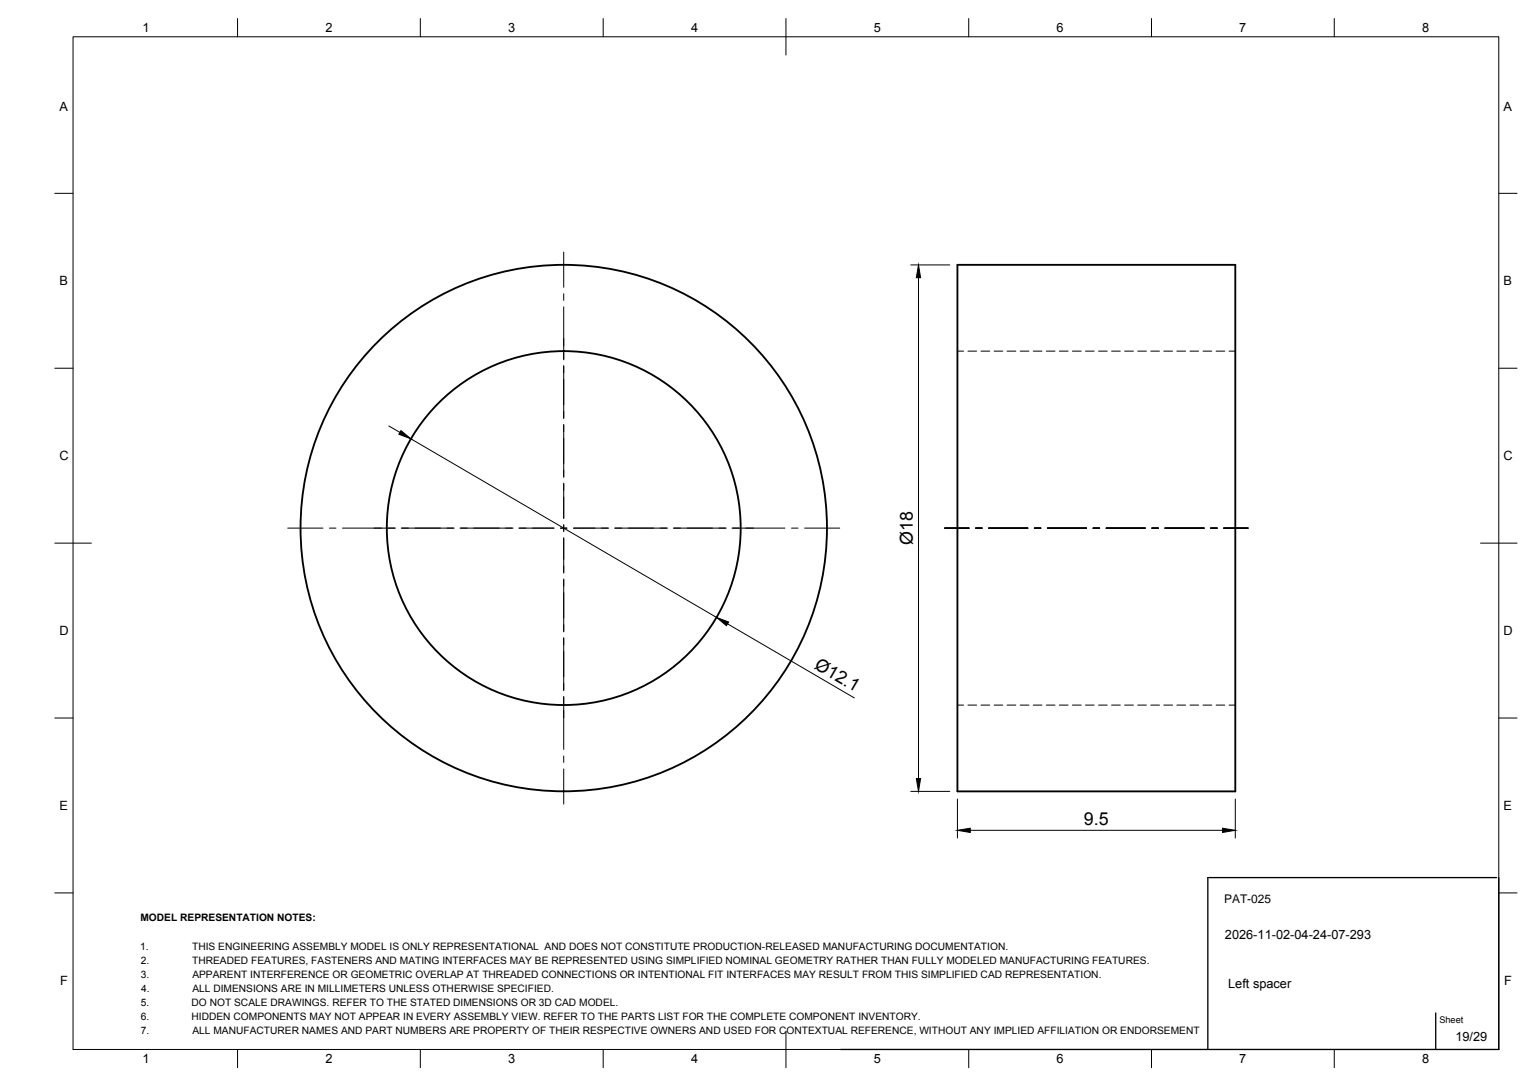
ISO-10303-21;
HEADER;
/* Generated by software containing ST-Developer
 * from STEP Tools, Inc. (www.steptools.com) 
 */

FILE_DESCRIPTION(
/* description */ ('Counter shaft with two pulleys and keyed hub'),
/* implementation_level */ '2;1');

FILE_NAME(
/* name */ 'Left spacer.step',
/* time_stamp */ '2026-10-27T10:46:10-07:00',
/* author */ (''),
/* organization */ (''),
/* preprocessor_version */ 'ST-DEVELOPER v20.2',
/* originating_system */ 'Autodesk Translation Framework v15.17.0.0',
/* authorisation */ '');

FILE_SCHEMA (('AUTOMOTIVE_DESIGN { 1 0 10303 214 3 1 1 }'));
ENDSEC;

DATA;
#10=MECHANICAL_DESIGN_GEOMETRIC_PRESENTATION_REPRESENTATION('',(#303),#10821);
#252=SHAPE_REPRESENTATION_RELATIONSHIP('SRR','None',#10940,#277);
#277=ADVANCED_BREP_SHAPE_REPRESENTATION('',(#328),#10808);
#303=STYLED_ITEM('',(#11149),#328);
#328=MANIFOLD_SOLID_BREP('Body1',#5587);
#395=FACE_BOUND('',#1085,.T.);
#396=FACE_BOUND('',#1087,.T.);
#515=PLANE('',#6121);
#516=PLANE('',#6122);
#713=FACE_OUTER_BOUND('',#1082,.T.);
#714=FACE_OUTER_BOUND('',#1083,.T.);
#715=FACE_OUTER_BOUND('',#1084,.T.);
#716=FACE_OUTER_BOUND('',#1086,.T.);
#1082=EDGE_LOOP('',(#4159,#4160,#4161,#4162));
#1083=EDGE_LOOP('',(#4163,#4164,#4165,#4166));
#1084=EDGE_LOOP('',(#4167));
#1085=EDGE_LOOP('',(#4168));
#1086=EDGE_LOOP('',(#4169));
#1087=EDGE_LOOP('',(#4170));
#1471=LINE('',#9333,#1860);
#1472=LINE('',#9339,#1861);
#1860=VECTOR('',#7203,0.605);
#1861=VECTOR('',#7210,0.9);
#2162=CIRCLE('',#6116,0.605);
#2163=CIRCLE('',#6117,0.605);
#2164=CIRCLE('',#6119,0.9);
#2165=CIRCLE('',#6120,0.9);
#2567=VERTEX_POINT('',#9330);
#2568=VERTEX_POINT('',#9332);
#2569=VERTEX_POINT('',#9336);
#2570=VERTEX_POINT('',#9338);
#3152=EDGE_CURVE('',#2567,#2567,#2162,.T.);
#3153=EDGE_CURVE('',#2567,#2568,#1471,.T.);
#3154=EDGE_CURVE('',#2568,#2568,#2163,.T.);
#3155=EDGE_CURVE('',#2569,#2569,#2164,.T.);
#3156=EDGE_CURVE('',#2569,#2570,#1472,.T.);
#3157=EDGE_CURVE('',#2570,#2570,#2165,.T.);
#4159=ORIENTED_EDGE('',*,*,#3152,.F.);
#4160=ORIENTED_EDGE('',*,*,#3153,.T.);
#4161=ORIENTED_EDGE('',*,*,#3154,.T.);
#4162=ORIENTED_EDGE('',*,*,#3153,.F.);
#4163=ORIENTED_EDGE('',*,*,#3155,.F.);
#4164=ORIENTED_EDGE('',*,*,#3156,.T.);
#4165=ORIENTED_EDGE('',*,*,#3157,.T.);
#4166=ORIENTED_EDGE('',*,*,#3156,.F.);
#4167=ORIENTED_EDGE('',*,*,#3155,.T.);
#4168=ORIENTED_EDGE('',*,*,#3152,.T.);
#4169=ORIENTED_EDGE('',*,*,#3157,.F.);
#4170=ORIENTED_EDGE('',*,*,#3154,.F.);
#5149=CYLINDRICAL_SURFACE('',#6115,0.605);
#5150=CYLINDRICAL_SURFACE('',#6118,0.9);
#5384=ADVANCED_FACE('',(#713),#5149,.F.);
#5385=ADVANCED_FACE('',(#714),#5150,.T.);
#5386=ADVANCED_FACE('',(#715,#395),#515,.T.);
#5387=ADVANCED_FACE('',(#716,#396),#516,.F.);
#5587=CLOSED_SHELL('',(#5384,#5385,#5386,#5387));
#6114=AXIS2_PLACEMENT_3D('',#9328,#7197,#7198);
#6115=AXIS2_PLACEMENT_3D('',#9329,#7199,#7200);
#6116=AXIS2_PLACEMENT_3D('',#9331,#7201,#7202);
#6117=AXIS2_PLACEMENT_3D('',#9334,#7204,#7205);
#6118=AXIS2_PLACEMENT_3D('',#9335,#7206,#7207);
#6119=AXIS2_PLACEMENT_3D('',#9337,#7208,#7209);
#6120=AXIS2_PLACEMENT_3D('',#9340,#7211,#7212);
#6121=AXIS2_PLACEMENT_3D('',#9341,#7213,#7214);
#6122=AXIS2_PLACEMENT_3D('',#9342,#7215,#7216);
#7197=DIRECTION('axis',(0.,0.,1.));
#7198=DIRECTION('refdir',(1.,0.,0.));
#7199=DIRECTION('center_axis',(0.,1.,0.));
#7200=DIRECTION('ref_axis',(1.,0.,0.));
#7201=DIRECTION('center_axis',(0.,-1.,0.));
#7202=DIRECTION('ref_axis',(1.,0.,0.));
#7203=DIRECTION('',(0.,-1.,0.));
#7204=DIRECTION('center_axis',(0.,-1.,0.));
#7205=DIRECTION('ref_axis',(1.,0.,0.));
#7206=DIRECTION('center_axis',(0.,1.,0.));
#7207=DIRECTION('ref_axis',(1.,0.,0.));
#7208=DIRECTION('center_axis',(0.,1.,0.));
#7209=DIRECTION('ref_axis',(1.,0.,0.));
#7210=DIRECTION('',(0.,-1.,0.));
#7211=DIRECTION('center_axis',(0.,1.,0.));
#7212=DIRECTION('ref_axis',(1.,0.,0.));
#7213=DIRECTION('center_axis',(0.,1.,0.));
#7214=DIRECTION('ref_axis',(1.,0.,0.));
#7215=DIRECTION('center_axis',(0.,1.,0.));
#7216=DIRECTION('ref_axis',(1.,0.,0.));
#9328=CARTESIAN_POINT('',(0.,0.,0.));
#9329=CARTESIAN_POINT('Origin',(0.,-3.45,4.53));
#9330=CARTESIAN_POINT('',(-0.605,-2.5,4.53));
#9331=CARTESIAN_POINT('Origin',(0.,-2.5,4.53));
#9332=CARTESIAN_POINT('',(-0.605,-3.45,4.53));
#9333=CARTESIAN_POINT('',(-0.605,-3.45,4.53));
#9334=CARTESIAN_POINT('Origin',(0.,-3.45,4.53));
#9335=CARTESIAN_POINT('Origin',(0.,-3.45,4.53));
#9336=CARTESIAN_POINT('',(-0.9,-2.5,4.53));
#9337=CARTESIAN_POINT('Origin',(0.,-2.5,4.53));
#9338=CARTESIAN_POINT('',(-0.9,-3.45,4.53));
#9339=CARTESIAN_POINT('',(-0.9,-3.45,4.53));
#9340=CARTESIAN_POINT('Origin',(0.,-3.45,4.53));
#9341=CARTESIAN_POINT('Origin',(0.,-2.5,4.53));
#9342=CARTESIAN_POINT('Origin',(0.,-3.45,4.53));
#10778=UNCERTAINTY_MEASURE_WITH_UNIT(LENGTH_MEASURE(0.001),#10822,
'DISTANCE_ACCURACY_VALUE',
'Maximum model space distance between geometric entities at asserted c
onnectivities');
#10791=UNCERTAINTY_MEASURE_WITH_UNIT(LENGTH_MEASURE(0.001),#10822,
'DISTANCE_ACCURACY_VALUE',
'Maximum model space distance between geometric entities at asserted c
onnectivities');
#10808=(
GEOMETRIC_REPRESENTATION_CONTEXT(3)
GLOBAL_UNCERTAINTY_ASSIGNED_CONTEXT((#10778))
GLOBAL_UNIT_ASSIGNED_CONTEXT((#10822,#10824,#10825))
REPRESENTATION_CONTEXT('','3D')
);
#10821=(
GEOMETRIC_REPRESENTATION_CONTEXT(3)
GLOBAL_UNCERTAINTY_ASSIGNED_CONTEXT((#10791))
GLOBAL_UNIT_ASSIGNED_CONTEXT((#10822,#10824,#10825))
REPRESENTATION_CONTEXT('','3D')
);
#10822=(
LENGTH_UNIT()
NAMED_UNIT(*)
SI_UNIT(.CENTI.,.METRE.)
);
#10824=(
NAMED_UNIT(*)
PLANE_ANGLE_UNIT()
SI_UNIT($,.RADIAN.)
);
#10825=(
NAMED_UNIT(*)
SI_UNIT($,.STERADIAN.)
SOLID_ANGLE_UNIT()
);
#10842=SHAPE_DEFINITION_REPRESENTATION(#10890,#10940);
#10890=PRODUCT_DEFINITION_SHAPE('',$,#10970);
#10940=SHAPE_REPRESENTATION('',(#6114),#10808);
#10953=PRODUCT_DEFINITION_CONTEXT('part definition',#11042,'design');
#10970=PRODUCT_DEFINITION('Left spacer','Left spacer',#10999,#10953);
#10999=PRODUCT_DEFINITION_FORMATION('',$,#11060);
#11042=APPLICATION_CONTEXT(
'Core Data for Automotive Mechanical Design Process');
#11043=PRODUCT_CONTEXT('part definition',#11042,'mechanical');
#11060=PRODUCT('Left spacer','Left spacer','Left spacer',(#11043));
#11143=COLOUR_RGB('Off White',0.89,0.88,0.83);
#11144=FILL_AREA_STYLE_COLOUR('',#11143);
#11145=FILL_AREA_STYLE('',(#11144));
#11146=SURFACE_STYLE_FILL_AREA(#11145);
#11147=SURFACE_SIDE_STYLE('',(#11146));
#11148=SURFACE_STYLE_USAGE(.BOTH.,#11147);
#11149=PRESENTATION_STYLE_ASSIGNMENT((#11148));
ENDSEC;
END-ISO-10303-21;
